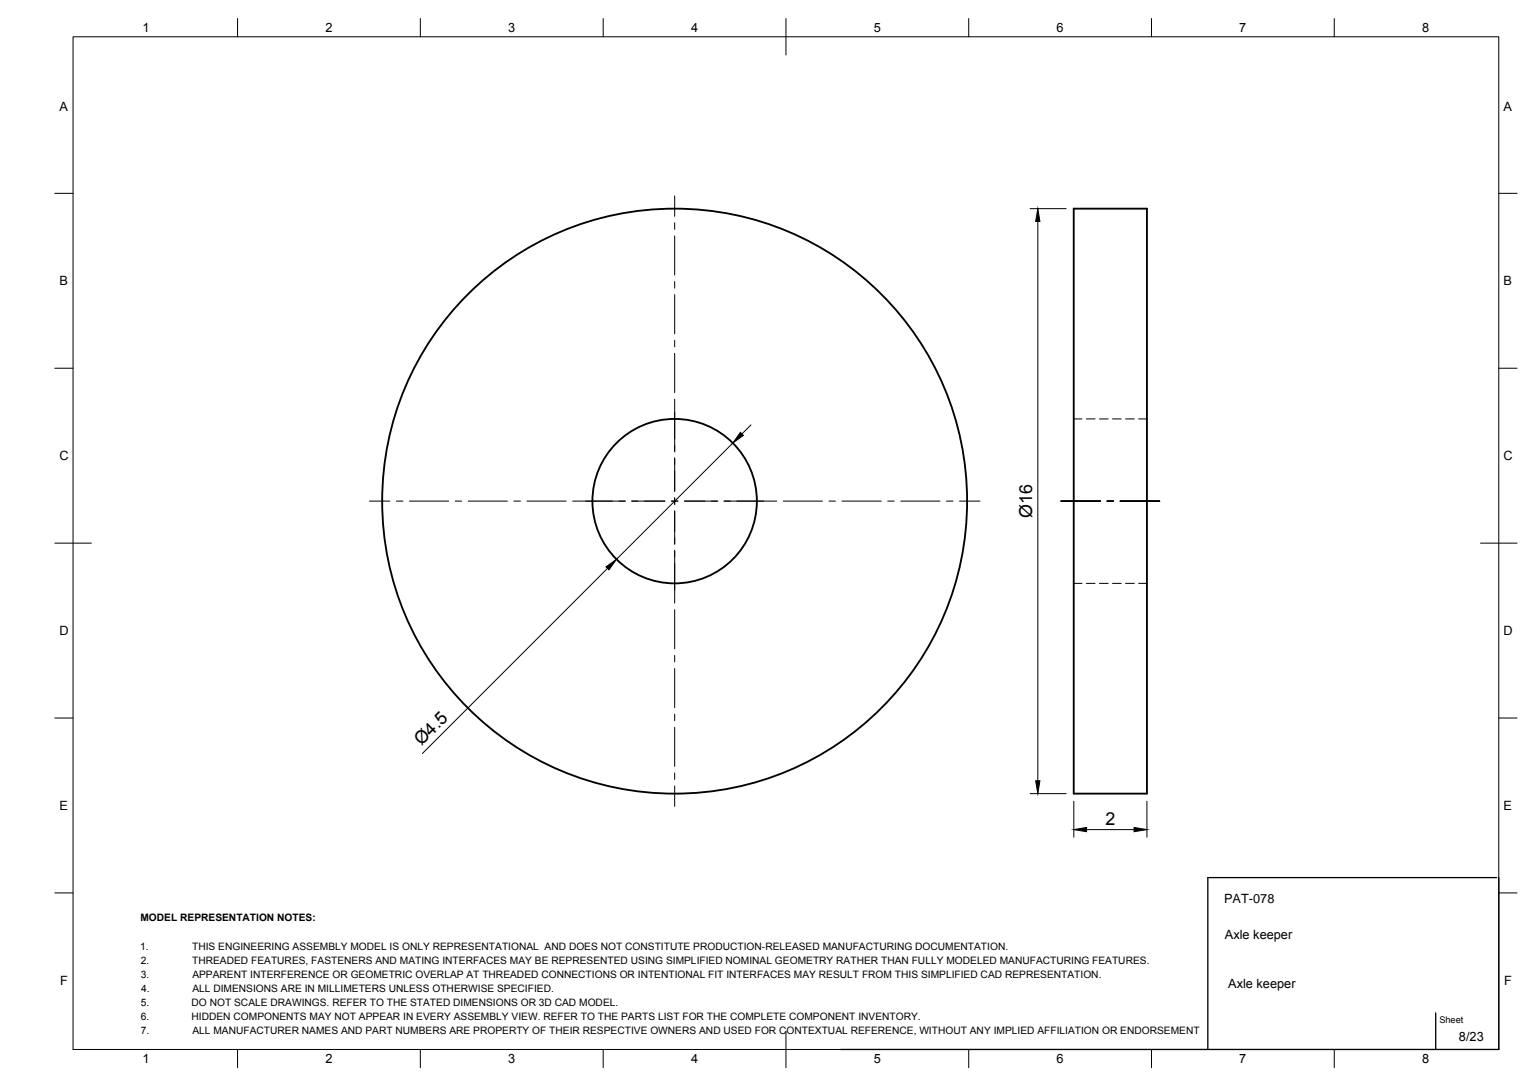
ISO-10303-21;
HEADER;
/* Generated by software containing ST-Developer
 * from STEP Tools, Inc. (www.steptools.com) 
 */

FILE_DESCRIPTION(
/* description */ ('Pedal-braked fixed caster'),
/* implementation_level */ '2;1');

FILE_NAME(
/* name */ 'Axle keeper.step',
/* time_stamp */ '2026-10-28T03:26:52-07:00',
/* author */ (''),
/* organization */ (''),
/* preprocessor_version */ 'ST-DEVELOPER v20.2',
/* originating_system */ 'Autodesk Translation Framework v15.17.0.0',
/* authorisation */ '');

FILE_SCHEMA (('AUTOMOTIVE_DESIGN { 1 0 10303 214 3 1 1 }'));
ENDSEC;

DATA;
#10=MECHANICAL_DESIGN_GEOMETRIC_PRESENTATION_REPRESENTATION('',(#209),#5734);
#175=SHAPE_REPRESENTATION_RELATIONSHIP('SRR','None',#5813,#192);
#192=ADVANCED_BREP_SHAPE_REPRESENTATION('',(#233),#5717);
#209=STYLED_ITEM('',(#5984),#233);
#233=MANIFOLD_SOLID_BREP('Body1',#2990);
#266=CYLINDRICAL_SURFACE('',#3285,0.225);
#267=CYLINDRICAL_SURFACE('',#3288,0.8);
#315=FACE_BOUND('',#730,.T.);
#316=FACE_BOUND('',#732,.T.);
#366=CIRCLE('',#3286,0.225);
#367=CIRCLE('',#3287,0.225);
#368=CIRCLE('',#3289,0.8);
#369=CIRCLE('',#3290,0.8);
#529=FACE_OUTER_BOUND('',#727,.T.);
#530=FACE_OUTER_BOUND('',#728,.T.);
#531=FACE_OUTER_BOUND('',#729,.T.);
#532=FACE_OUTER_BOUND('',#731,.T.);
#727=EDGE_LOOP('',(#2198,#2199,#2200,#2201));
#728=EDGE_LOOP('',(#2202,#2203,#2204,#2205));
#729=EDGE_LOOP('',(#2206));
#730=EDGE_LOOP('',(#2207));
#731=EDGE_LOOP('',(#2208));
#732=EDGE_LOOP('',(#2209));
#980=LINE('',#4773,#1192);
#981=LINE('',#4779,#1193);
#1192=VECTOR('',#3838,0.225);
#1193=VECTOR('',#3845,0.8);
#1387=VERTEX_POINT('',#4770);
#1388=VERTEX_POINT('',#4772);
#1389=VERTEX_POINT('',#4776);
#1390=VERTEX_POINT('',#4778);
#1689=EDGE_CURVE('',#1387,#1387,#366,.T.);
#1690=EDGE_CURVE('',#1387,#1388,#980,.T.);
#1691=EDGE_CURVE('',#1388,#1388,#367,.T.);
#1692=EDGE_CURVE('',#1389,#1389,#368,.T.);
#1693=EDGE_CURVE('',#1389,#1390,#981,.T.);
#1694=EDGE_CURVE('',#1390,#1390,#369,.T.);
#2198=ORIENTED_EDGE('',*,*,#1689,.F.);
#2199=ORIENTED_EDGE('',*,*,#1690,.T.);
#2200=ORIENTED_EDGE('',*,*,#1691,.T.);
#2201=ORIENTED_EDGE('',*,*,#1690,.F.);
#2202=ORIENTED_EDGE('',*,*,#1692,.F.);
#2203=ORIENTED_EDGE('',*,*,#1693,.T.);
#2204=ORIENTED_EDGE('',*,*,#1694,.T.);
#2205=ORIENTED_EDGE('',*,*,#1693,.F.);
#2206=ORIENTED_EDGE('',*,*,#1692,.T.);
#2207=ORIENTED_EDGE('',*,*,#1689,.T.);
#2208=ORIENTED_EDGE('',*,*,#1694,.F.);
#2209=ORIENTED_EDGE('',*,*,#1691,.F.);
#2740=PLANE('',#3291);
#2741=PLANE('',#3292);
#2862=ADVANCED_FACE('',(#529),#266,.F.);
#2863=ADVANCED_FACE('',(#530),#267,.T.);
#2864=ADVANCED_FACE('',(#531,#315),#2740,.T.);
#2865=ADVANCED_FACE('',(#532,#316),#2741,.F.);
#2990=CLOSED_SHELL('',(#2862,#2863,#2864,#2865));
#3284=AXIS2_PLACEMENT_3D('',#4768,#3832,#3833);
#3285=AXIS2_PLACEMENT_3D('',#4769,#3834,#3835);
#3286=AXIS2_PLACEMENT_3D('',#4771,#3836,#3837);
#3287=AXIS2_PLACEMENT_3D('',#4774,#3839,#3840);
#3288=AXIS2_PLACEMENT_3D('',#4775,#3841,#3842);
#3289=AXIS2_PLACEMENT_3D('',#4777,#3843,#3844);
#3290=AXIS2_PLACEMENT_3D('',#4780,#3846,#3847);
#3291=AXIS2_PLACEMENT_3D('',#4781,#3848,#3849);
#3292=AXIS2_PLACEMENT_3D('',#4782,#3850,#3851);
#3832=DIRECTION('axis',(0.,0.,1.));
#3833=DIRECTION('refdir',(1.,0.,0.));
#3834=DIRECTION('center_axis',(0.,1.,0.));
#3835=DIRECTION('ref_axis',(1.,0.,0.));
#3836=DIRECTION('center_axis',(0.,-1.,0.));
#3837=DIRECTION('ref_axis',(1.,0.,0.));
#3838=DIRECTION('',(0.,-1.,0.));
#3839=DIRECTION('center_axis',(0.,-1.,0.));
#3840=DIRECTION('ref_axis',(1.,0.,0.));
#3841=DIRECTION('center_axis',(0.,1.,0.));
#3842=DIRECTION('ref_axis',(1.,0.,0.));
#3843=DIRECTION('center_axis',(0.,1.,0.));
#3844=DIRECTION('ref_axis',(1.,0.,0.));
#3845=DIRECTION('',(0.,-1.,0.));
#3846=DIRECTION('center_axis',(0.,1.,0.));
#3847=DIRECTION('ref_axis',(1.,0.,0.));
#3848=DIRECTION('center_axis',(0.,1.,0.));
#3849=DIRECTION('ref_axis',(1.,0.,0.));
#3850=DIRECTION('center_axis',(0.,1.,0.));
#3851=DIRECTION('ref_axis',(1.,0.,0.));
#4768=CARTESIAN_POINT('',(0.,0.,0.));
#4769=CARTESIAN_POINT('Origin',(0.,2.2,4.));
#4770=CARTESIAN_POINT('',(-0.225,2.4,4.));
#4771=CARTESIAN_POINT('Origin',(0.,2.4,4.));
#4772=CARTESIAN_POINT('',(-0.225,2.2,4.));
#4773=CARTESIAN_POINT('',(-0.225,2.2,4.));
#4774=CARTESIAN_POINT('Origin',(0.,2.2,4.));
#4775=CARTESIAN_POINT('Origin',(0.,2.2,4.));
#4776=CARTESIAN_POINT('',(-0.8,2.4,4.));
#4777=CARTESIAN_POINT('Origin',(0.,2.4,4.));
#4778=CARTESIAN_POINT('',(-0.8,2.2,4.));
#4779=CARTESIAN_POINT('',(-0.8,2.2,4.));
#4780=CARTESIAN_POINT('Origin',(0.,2.2,4.));
#4781=CARTESIAN_POINT('Origin',(0.,2.4,4.));
#4782=CARTESIAN_POINT('Origin',(0.,2.2,4.));
#5694=UNCERTAINTY_MEASURE_WITH_UNIT(LENGTH_MEASURE(0.001),#5735,
'DISTANCE_ACCURACY_VALUE',
'Maximum model space distance between geometric entities at asserted c
onnectivities');
#5711=UNCERTAINTY_MEASURE_WITH_UNIT(LENGTH_MEASURE(0.001),#5735,
'DISTANCE_ACCURACY_VALUE',
'Maximum model space distance between geometric entities at asserted c
onnectivities');
#5717=(
GEOMETRIC_REPRESENTATION_CONTEXT(3)
GLOBAL_UNCERTAINTY_ASSIGNED_CONTEXT((#5694))
GLOBAL_UNIT_ASSIGNED_CONTEXT((#5735,#5737,#5738))
REPRESENTATION_CONTEXT('','3D')
);
#5734=(
GEOMETRIC_REPRESENTATION_CONTEXT(3)
GLOBAL_UNCERTAINTY_ASSIGNED_CONTEXT((#5711))
GLOBAL_UNIT_ASSIGNED_CONTEXT((#5735,#5737,#5738))
REPRESENTATION_CONTEXT('','3D')
);
#5735=(
LENGTH_UNIT()
NAMED_UNIT(*)
SI_UNIT(.CENTI.,.METRE.)
);
#5737=(
NAMED_UNIT(*)
PLANE_ANGLE_UNIT()
SI_UNIT($,.RADIAN.)
);
#5738=(
NAMED_UNIT(*)
SI_UNIT($,.STERADIAN.)
SOLID_ANGLE_UNIT()
);
#5744=SHAPE_DEFINITION_REPRESENTATION(#5766,#5813);
#5766=PRODUCT_DEFINITION_SHAPE('',$,#5836);
#5813=SHAPE_REPRESENTATION('',(#3284),#5717);
#5830=PRODUCT_DEFINITION_CONTEXT('part definition',#5898,'design');
#5836=PRODUCT_DEFINITION('Axle keeper','Axle keeper',#5858,#5830);
#5858=PRODUCT_DEFINITION_FORMATION('',$,#5905);
#5898=APPLICATION_CONTEXT(
'Core Data for Automotive Mechanical Design Process');
#5899=PRODUCT_CONTEXT('part definition',#5898,'mechanical');
#5905=PRODUCT('Axle keeper','Axle keeper','Axle keeper',(#5899));
#5978=COLOUR_RGB('Grey',0.48,0.52,0.57);
#5979=FILL_AREA_STYLE_COLOUR('',#5978);
#5980=FILL_AREA_STYLE('',(#5979));
#5981=SURFACE_STYLE_FILL_AREA(#5980);
#5982=SURFACE_SIDE_STYLE('',(#5981));
#5983=SURFACE_STYLE_USAGE(.BOTH.,#5982);
#5984=PRESENTATION_STYLE_ASSIGNMENT((#5983));
ENDSEC;
END-ISO-10303-21;
